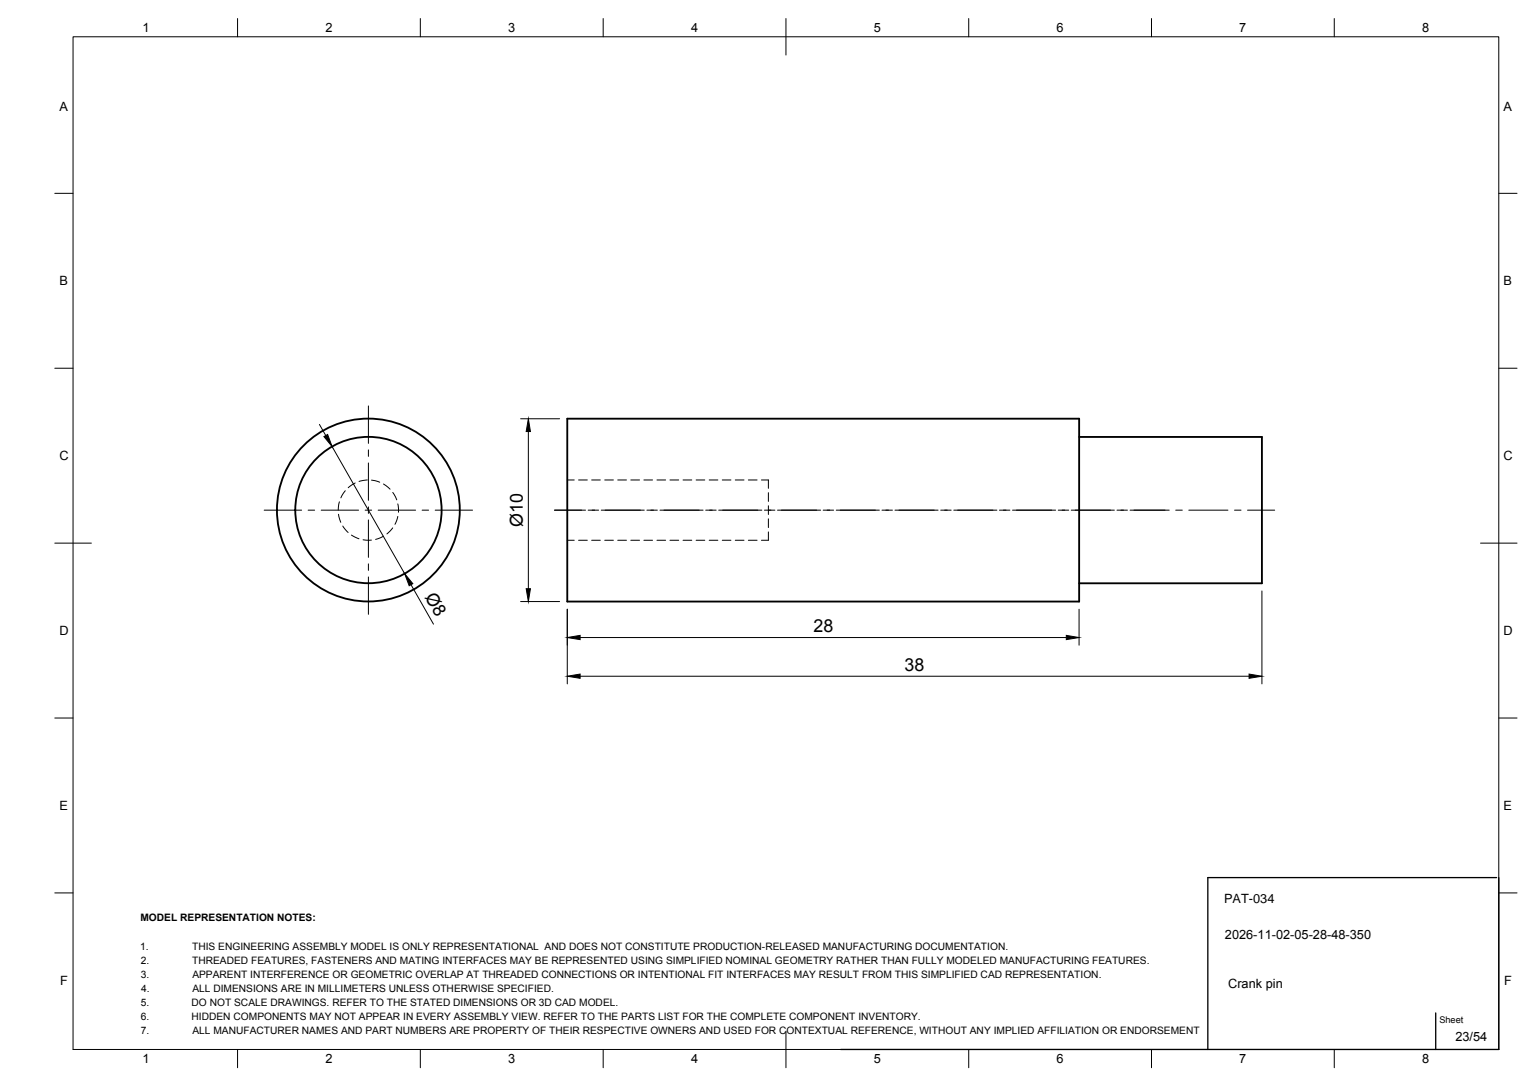
ISO-10303-21;
HEADER;
/* Generated by software containing ST-Developer
 * from STEP Tools, Inc. (www.steptools.com) 
 */

FILE_DESCRIPTION(
/* description */ ('Fatigue rig crank-slider'),
/* implementation_level */ '2;1');

FILE_NAME(
/* name */ 'Crank pin.step',
/* time_stamp */ '2026-10-28T03:24:50-07:00',
/* author */ (''),
/* organization */ (''),
/* preprocessor_version */ 'ST-DEVELOPER v20.2',
/* originating_system */ 'Autodesk Translation Framework v15.17.0.0',
/* authorisation */ '');

FILE_SCHEMA (('AUTOMOTIVE_DESIGN { 1 0 10303 214 3 1 1 }'));
ENDSEC;

DATA;
#10=MECHANICAL_DESIGN_GEOMETRIC_PRESENTATION_REPRESENTATION('',(#609),#16911);
#508=SHAPE_REPRESENTATION_RELATIONSHIP('SRR','None',#17149,#558);
#558=ADVANCED_BREP_SHAPE_REPRESENTATION('',(#666),#16878);
#609=STYLED_ITEM('',(#17487),#666);
#666=MANIFOLD_SOLID_BREP('Body1',#8902);
#833=FACE_BOUND('',#2136,.T.);
#834=FACE_BOUND('',#2139,.T.);
#1053=PLANE('',#9987);
#1054=PLANE('',#9988);
#1055=PLANE('',#9993);
#1056=PLANE('',#9996);
#1477=FACE_OUTER_BOUND('',#2133,.T.);
#1478=FACE_OUTER_BOUND('',#2134,.T.);
#1479=FACE_OUTER_BOUND('',#2135,.T.);
#1480=FACE_OUTER_BOUND('',#2137,.T.);
#1481=FACE_OUTER_BOUND('',#2138,.T.);
#1482=FACE_OUTER_BOUND('',#2140,.T.);
#1483=FACE_OUTER_BOUND('',#2141,.T.);
#2133=EDGE_LOOP('',(#7104,#7105,#7106,#7107));
#2134=EDGE_LOOP('',(#7108));
#2135=EDGE_LOOP('',(#7109));
#2136=EDGE_LOOP('',(#7110));
#2137=EDGE_LOOP('',(#7111,#7112,#7113,#7114));
#2138=EDGE_LOOP('',(#7115));
#2139=EDGE_LOOP('',(#7116));
#2140=EDGE_LOOP('',(#7117,#7118,#7119,#7120));
#2141=EDGE_LOOP('',(#7121));
#2775=LINE('',#15160,#3421);
#2776=LINE('',#15171,#3422);
#2777=LINE('',#15175,#3423);
#3421=VECTOR('',#11867,0.165);
#3422=VECTOR('',#11882,0.5);
#3423=VECTOR('',#11887,0.4);
#3955=CIRCLE('',#9985,0.165);
#3956=CIRCLE('',#9986,0.165);
#3957=CIRCLE('',#9989,0.5);
#3958=CIRCLE('',#9990,0.4);
#3959=CIRCLE('',#9992,0.5);
#3960=CIRCLE('',#9995,0.4);
#4527=VERTEX_POINT('',#15157);
#4528=VERTEX_POINT('',#15159);
#4529=VERTEX_POINT('',#15164);
#4530=VERTEX_POINT('',#15166);
#4531=VERTEX_POINT('',#15169);
#4532=VERTEX_POINT('',#15174);
#5450=EDGE_CURVE('',#4527,#4527,#3955,.T.);
#5451=EDGE_CURVE('',#4527,#4528,#2775,.T.);
#5452=EDGE_CURVE('',#4528,#4528,#3956,.T.);
#5453=EDGE_CURVE('',#4529,#4529,#3957,.T.);
#5454=EDGE_CURVE('',#4530,#4530,#3958,.T.);
#5455=EDGE_CURVE('',#4531,#4531,#3959,.T.);
#5456=EDGE_CURVE('',#4531,#4529,#2776,.T.);
#5457=EDGE_CURVE('',#4530,#4532,#2777,.T.);
#5458=EDGE_CURVE('',#4532,#4532,#3960,.T.);
#7104=ORIENTED_EDGE('',*,*,#5450,.F.);
#7105=ORIENTED_EDGE('',*,*,#5451,.T.);
#7106=ORIENTED_EDGE('',*,*,#5452,.F.);
#7107=ORIENTED_EDGE('',*,*,#5451,.F.);
#7108=ORIENTED_EDGE('',*,*,#5450,.T.);
#7109=ORIENTED_EDGE('',*,*,#5453,.F.);
#7110=ORIENTED_EDGE('',*,*,#5454,.T.);
#7111=ORIENTED_EDGE('',*,*,#5455,.F.);
#7112=ORIENTED_EDGE('',*,*,#5456,.T.);
#7113=ORIENTED_EDGE('',*,*,#5453,.T.);
#7114=ORIENTED_EDGE('',*,*,#5456,.F.);
#7115=ORIENTED_EDGE('',*,*,#5455,.T.);
#7116=ORIENTED_EDGE('',*,*,#5452,.T.);
#7117=ORIENTED_EDGE('',*,*,#5454,.F.);
#7118=ORIENTED_EDGE('',*,*,#5457,.T.);
#7119=ORIENTED_EDGE('',*,*,#5458,.T.);
#7120=ORIENTED_EDGE('',*,*,#5457,.F.);
#7121=ORIENTED_EDGE('',*,*,#5458,.F.);
#8291=CYLINDRICAL_SURFACE('',#9984,0.165);
#8292=CYLINDRICAL_SURFACE('',#9991,0.5);
#8293=CYLINDRICAL_SURFACE('',#9994,0.4);
#8615=ADVANCED_FACE('',(#1477),#8291,.F.);
#8616=ADVANCED_FACE('',(#1478),#1053,.T.);
#8617=ADVANCED_FACE('',(#1479,#833),#1054,.F.);
#8618=ADVANCED_FACE('',(#1480),#8292,.T.);
#8619=ADVANCED_FACE('',(#1481,#834),#1055,.T.);
#8620=ADVANCED_FACE('',(#1482),#8293,.T.);
#8621=ADVANCED_FACE('',(#1483),#1056,.F.);
#8902=CLOSED_SHELL('',(#8615,#8616,#8617,#8618,#8619,#8620,#8621));
#9983=AXIS2_PLACEMENT_3D('',#15155,#11861,#11862);
#9984=AXIS2_PLACEMENT_3D('',#15156,#11863,#11864);
#9985=AXIS2_PLACEMENT_3D('',#15158,#11865,#11866);
#9986=AXIS2_PLACEMENT_3D('',#15161,#11868,#11869);
#9987=AXIS2_PLACEMENT_3D('',#15162,#11870,#11871);
#9988=AXIS2_PLACEMENT_3D('',#15163,#11872,#11873);
#9989=AXIS2_PLACEMENT_3D('',#15165,#11874,#11875);
#9990=AXIS2_PLACEMENT_3D('',#15167,#11876,#11877);
#9991=AXIS2_PLACEMENT_3D('',#15168,#11878,#11879);
#9992=AXIS2_PLACEMENT_3D('',#15170,#11880,#11881);
#9993=AXIS2_PLACEMENT_3D('',#15172,#11883,#11884);
#9994=AXIS2_PLACEMENT_3D('',#15173,#11885,#11886);
#9995=AXIS2_PLACEMENT_3D('',#15176,#11888,#11889);
#9996=AXIS2_PLACEMENT_3D('',#15177,#11890,#11891);
#11861=DIRECTION('axis',(0.,0.,1.));
#11862=DIRECTION('refdir',(1.,0.,0.));
#11863=DIRECTION('center_axis',(0.,1.,0.));
#11864=DIRECTION('ref_axis',(1.,0.,0.));
#11865=DIRECTION('center_axis',(0.,1.,0.));
#11866=DIRECTION('ref_axis',(1.,0.,0.));
#11867=DIRECTION('',(0.,1.,0.));
#11868=DIRECTION('center_axis',(0.,-1.,0.));
#11869=DIRECTION('ref_axis',(1.,0.,0.));
#11870=DIRECTION('center_axis',(0.,1.,0.));
#11871=DIRECTION('ref_axis',(1.,0.,0.));
#11872=DIRECTION('center_axis',(0.,1.,0.));
#11873=DIRECTION('ref_axis',(1.,0.,0.));
#11874=DIRECTION('center_axis',(0.,1.,0.));
#11875=DIRECTION('ref_axis',(1.,0.,0.));
#11876=DIRECTION('center_axis',(0.,1.,0.));
#11877=DIRECTION('ref_axis',(1.,0.,0.));
#11878=DIRECTION('center_axis',(0.,1.,0.));
#11879=DIRECTION('ref_axis',(1.,0.,0.));
#11880=DIRECTION('center_axis',(0.,1.,0.));
#11881=DIRECTION('ref_axis',(1.,0.,0.));
#11882=DIRECTION('',(0.,-1.,0.));
#11883=DIRECTION('center_axis',(0.,1.,0.));
#11884=DIRECTION('ref_axis',(1.,0.,0.));
#11885=DIRECTION('center_axis',(0.,1.,0.));
#11886=DIRECTION('ref_axis',(1.,0.,0.));
#11887=DIRECTION('',(0.,-1.,0.));
#11888=DIRECTION('center_axis',(0.,1.,0.));
#11889=DIRECTION('ref_axis',(1.,0.,0.));
#11890=DIRECTION('center_axis',(0.,1.,0.));
#11891=DIRECTION('ref_axis',(1.,0.,0.));
#15155=CARTESIAN_POINT('',(0.,0.,0.));
#15156=CARTESIAN_POINT('Origin',(1.,3.7,12.));
#15157=CARTESIAN_POINT('',(0.835,3.7,12.));
#15158=CARTESIAN_POINT('Origin',(1.,3.7,12.));
#15159=CARTESIAN_POINT('',(0.835,4.8,12.));
#15160=CARTESIAN_POINT('',(0.835,3.7,12.));
#15161=CARTESIAN_POINT('Origin',(1.,4.8,12.));
#15162=CARTESIAN_POINT('Origin',(1.,3.7,12.));
#15163=CARTESIAN_POINT('Origin',(1.,2.,12.));
#15164=CARTESIAN_POINT('',(0.5,2.,12.));
#15165=CARTESIAN_POINT('Origin',(1.,2.,12.));
#15166=CARTESIAN_POINT('',(0.6,2.,12.));
#15167=CARTESIAN_POINT('Origin',(1.,2.,12.));
#15168=CARTESIAN_POINT('Origin',(1.,2.,12.));
#15169=CARTESIAN_POINT('',(0.5,4.8,12.));
#15170=CARTESIAN_POINT('Origin',(1.,4.8,12.));
#15171=CARTESIAN_POINT('',(0.5,2.,12.));
#15172=CARTESIAN_POINT('Origin',(1.,4.8,12.));
#15173=CARTESIAN_POINT('Origin',(1.,1.,12.));
#15174=CARTESIAN_POINT('',(0.6,1.,12.));
#15175=CARTESIAN_POINT('',(0.6,1.,12.));
#15176=CARTESIAN_POINT('Origin',(1.,1.,12.));
#15177=CARTESIAN_POINT('Origin',(1.,1.,12.));
#16819=UNCERTAINTY_MEASURE_WITH_UNIT(LENGTH_MEASURE(0.001),#16912,
'DISTANCE_ACCURACY_VALUE',
'Maximum model space distance between geometric entities at asserted c
onnectivities');
#16852=UNCERTAINTY_MEASURE_WITH_UNIT(LENGTH_MEASURE(0.001),#16912,
'DISTANCE_ACCURACY_VALUE',
'Maximum model space distance between geometric entities at asserted c
onnectivities');
#16878=(
GEOMETRIC_REPRESENTATION_CONTEXT(3)
GLOBAL_UNCERTAINTY_ASSIGNED_CONTEXT((#16819))
GLOBAL_UNIT_ASSIGNED_CONTEXT((#16912,#16914,#16915))
REPRESENTATION_CONTEXT('','3D')
);
#16911=(
GEOMETRIC_REPRESENTATION_CONTEXT(3)
GLOBAL_UNCERTAINTY_ASSIGNED_CONTEXT((#16852))
GLOBAL_UNIT_ASSIGNED_CONTEXT((#16912,#16914,#16915))
REPRESENTATION_CONTEXT('','3D')
);
#16912=(
LENGTH_UNIT()
NAMED_UNIT(*)
SI_UNIT(.CENTI.,.METRE.)
);
#16914=(
NAMED_UNIT(*)
PLANE_ANGLE_UNIT()
SI_UNIT($,.RADIAN.)
);
#16915=(
NAMED_UNIT(*)
SI_UNIT($,.STERADIAN.)
SOLID_ANGLE_UNIT()
);
#16941=SHAPE_DEFINITION_REPRESENTATION(#17001,#17149);
#17001=PRODUCT_DEFINITION_SHAPE('',$,#17208);
#17149=SHAPE_REPRESENTATION('',(#9983),#16878);
#17182=PRODUCT_DEFINITION_CONTEXT('part definition',#17358,'design');
#17208=PRODUCT_DEFINITION('Crank pin','Crank pin',#17266,#17182);
#17266=PRODUCT_DEFINITION_FORMATION('',$,#17385);
#17358=APPLICATION_CONTEXT(
'Core Data for Automotive Mechanical Design Process');
#17359=PRODUCT_CONTEXT('part definition',#17358,'mechanical');
#17385=PRODUCT('Crank pin','Crank pin','Crank pin',(#17359));
#17481=COLOUR_RGB('Grey',0.48,0.52,0.57);
#17482=FILL_AREA_STYLE_COLOUR('',#17481);
#17483=FILL_AREA_STYLE('',(#17482));
#17484=SURFACE_STYLE_FILL_AREA(#17483);
#17485=SURFACE_SIDE_STYLE('',(#17484));
#17486=SURFACE_STYLE_USAGE(.BOTH.,#17485);
#17487=PRESENTATION_STYLE_ASSIGNMENT((#17486));
ENDSEC;
END-ISO-10303-21;
